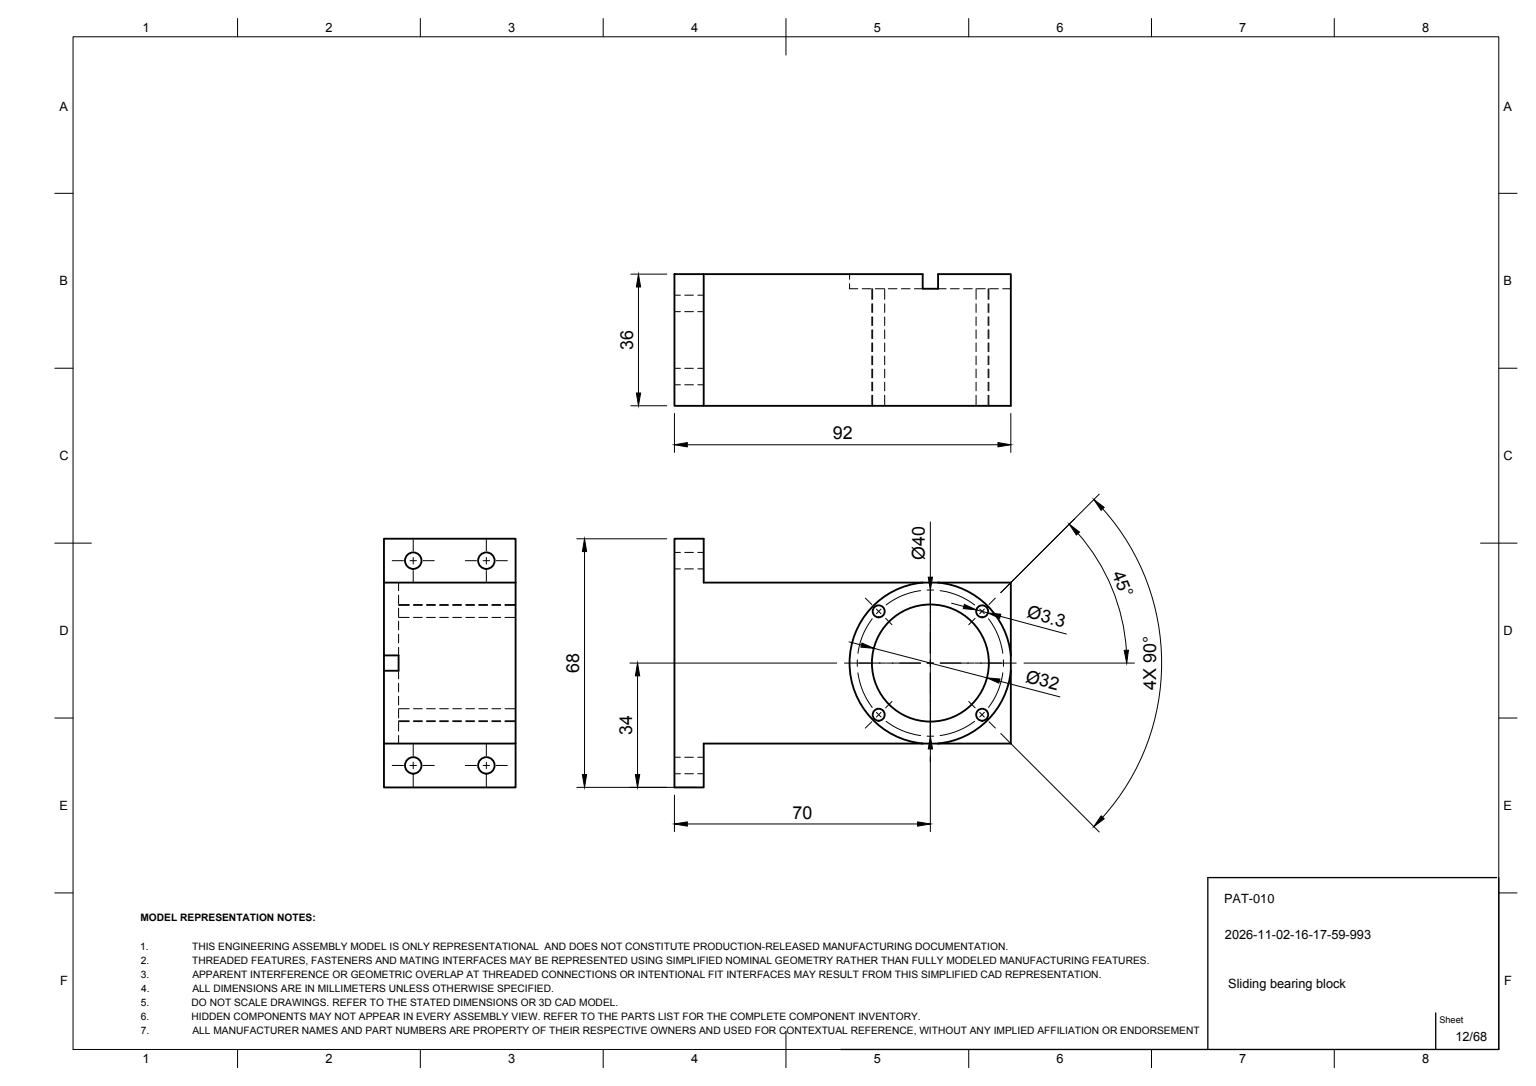
ISO-10303-21;
HEADER;
/* Generated by software containing ST-Developer
 * from STEP Tools, Inc. (www.steptools.com) 
 */

FILE_DESCRIPTION(
/* description */ ('Belt conveyor head drive unit'),
/* implementation_level */ '2;1');

FILE_NAME(
/* name */ 'Sliding bearing block.step',
/* time_stamp */ '2026-10-28T03:26:19-07:00',
/* author */ (''),
/* organization */ (''),
/* preprocessor_version */ 'ST-DEVELOPER v20.2',
/* originating_system */ 'Autodesk Translation Framework v15.17.0.0',
/* authorisation */ '');

FILE_SCHEMA (('AUTOMOTIVE_DESIGN { 1 0 10303 214 3 1 1 }'));
ENDSEC;

DATA;
#10=MECHANICAL_DESIGN_GEOMETRIC_PRESENTATION_REPRESENTATION('',(#854),#27069);
#716=SHAPE_REPRESENTATION_RELATIONSHIP('SRR','None',#27360,#785);
#785=ADVANCED_BREP_SHAPE_REPRESENTATION('',(#939),#27002);
#854=STYLED_ITEM('',(#27797),#939);
#939=MANIFOLD_SOLID_BREP('Body1',#13719);
#1058=FACE_BOUND('',#2593,.T.);
#1059=FACE_BOUND('',#2594,.T.);
#1060=FACE_BOUND('',#2595,.T.);
#1061=FACE_BOUND('',#2596,.T.);
#1062=FACE_BOUND('',#2597,.T.);
#1063=FACE_BOUND('',#2613,.T.);
#1064=FACE_BOUND('',#2614,.T.);
#1065=FACE_BOUND('',#2616,.T.);
#1066=FACE_BOUND('',#2617,.T.);
#1067=FACE_BOUND('',#2621,.T.);
#1068=FACE_BOUND('',#2622,.T.);
#1069=FACE_BOUND('',#2623,.T.);
#1070=FACE_BOUND('',#2624,.T.);
#1071=FACE_BOUND('',#2625,.T.);
#1072=FACE_BOUND('',#2629,.T.);
#1073=FACE_BOUND('',#2630,.T.);
#1074=FACE_BOUND('',#2631,.T.);
#1075=FACE_BOUND('',#2632,.T.);
#1335=PLANE('',#14799);
#1336=PLANE('',#14808);
#1337=PLANE('',#14809);
#1338=PLANE('',#14810);
#1339=PLANE('',#14811);
#1340=PLANE('',#14834);
#1341=PLANE('',#14835);
#1342=PLANE('',#14836);
#1343=PLANE('',#14837);
#1344=PLANE('',#14838);
#1345=PLANE('',#14839);
#1346=PLANE('',#14840);
#1347=PLANE('',#14841);
#1744=FACE_OUTER_BOUND('',#2590,.T.);
#1745=FACE_OUTER_BOUND('',#2591,.T.);
#1746=FACE_OUTER_BOUND('',#2592,.T.);
#1747=FACE_OUTER_BOUND('',#2598,.T.);
#1748=FACE_OUTER_BOUND('',#2599,.T.);
#1749=FACE_OUTER_BOUND('',#2600,.T.);
#1750=FACE_OUTER_BOUND('',#2601,.T.);
#1751=FACE_OUTER_BOUND('',#2602,.T.);
#1752=FACE_OUTER_BOUND('',#2603,.T.);
#1753=FACE_OUTER_BOUND('',#2604,.T.);
#1754=FACE_OUTER_BOUND('',#2605,.T.);
#1755=FACE_OUTER_BOUND('',#2606,.T.);
#1756=FACE_OUTER_BOUND('',#2607,.T.);
#1757=FACE_OUTER_BOUND('',#2608,.T.);
#1758=FACE_OUTER_BOUND('',#2609,.T.);
#1759=FACE_OUTER_BOUND('',#2610,.T.);
#1760=FACE_OUTER_BOUND('',#2611,.T.);
#1761=FACE_OUTER_BOUND('',#2612,.T.);
#1762=FACE_OUTER_BOUND('',#2615,.T.);
#1763=FACE_OUTER_BOUND('',#2618,.T.);
#1764=FACE_OUTER_BOUND('',#2619,.T.);
#1765=FACE_OUTER_BOUND('',#2620,.T.);
#1766=FACE_OUTER_BOUND('',#2626,.T.);
#1767=FACE_OUTER_BOUND('',#2627,.T.);
#1768=FACE_OUTER_BOUND('',#2628,.T.);
#2590=EDGE_LOOP('',(#9456,#9457,#9458,#9459));
#2591=EDGE_LOOP('',(#9460,#9461,#9462,#9463));
#2592=EDGE_LOOP('',(#9464,#9465,#9466,#9467,#9468,#9469));
#2593=EDGE_LOOP('',(#9470));
#2594=EDGE_LOOP('',(#9471));
#2595=EDGE_LOOP('',(#9472));
#2596=EDGE_LOOP('',(#9473));
#2597=EDGE_LOOP('',(#9474));
#2598=EDGE_LOOP('',(#9475,#9476,#9477,#9478));
#2599=EDGE_LOOP('',(#9479,#9480,#9481,#9482,#9483,#9484,#9485,#9486));
#2600=EDGE_LOOP('',(#9487,#9488,#9489,#9490,#9491,#9492,#9493,#9494));
#2601=EDGE_LOOP('',(#9495,#9496,#9497));
#2602=EDGE_LOOP('',(#9498,#9499,#9500));
#2603=EDGE_LOOP('',(#9501,#9502,#9503,#9504));
#2604=EDGE_LOOP('',(#9505,#9506,#9507,#9508));
#2605=EDGE_LOOP('',(#9509,#9510,#9511,#9512));
#2606=EDGE_LOOP('',(#9513,#9514,#9515,#9516));
#2607=EDGE_LOOP('',(#9517,#9518,#9519,#9520));
#2608=EDGE_LOOP('',(#9521,#9522,#9523,#9524));
#2609=EDGE_LOOP('',(#9525,#9526,#9527,#9528));
#2610=EDGE_LOOP('',(#9529,#9530,#9531,#9532));
#2611=EDGE_LOOP('',(#9533,#9534,#9535,#9536));
#2612=EDGE_LOOP('',(#9537,#9538,#9539,#9540));
#2613=EDGE_LOOP('',(#9541));
#2614=EDGE_LOOP('',(#9542));
#2615=EDGE_LOOP('',(#9543,#9544,#9545,#9546));
#2616=EDGE_LOOP('',(#9547));
#2617=EDGE_LOOP('',(#9548));
#2618=EDGE_LOOP('',(#9549,#9550,#9551,#9552));
#2619=EDGE_LOOP('',(#9553,#9554,#9555,#9556));
#2620=EDGE_LOOP('',(#9557,#9558,#9559,#9560,#9561,#9562,#9563,#9564));
#2621=EDGE_LOOP('',(#9565));
#2622=EDGE_LOOP('',(#9566));
#2623=EDGE_LOOP('',(#9567));
#2624=EDGE_LOOP('',(#9568));
#2625=EDGE_LOOP('',(#9569));
#2626=EDGE_LOOP('',(#9570,#9571,#9572,#9573,#9574,#9575,#9576,#9577));
#2627=EDGE_LOOP('',(#9578,#9579,#9580,#9581,#9582,#9583,#9584,#9585));
#2628=EDGE_LOOP('',(#9586,#9587,#9588,#9589));
#2629=EDGE_LOOP('',(#9590));
#2630=EDGE_LOOP('',(#9591));
#2631=EDGE_LOOP('',(#9592));
#2632=EDGE_LOOP('',(#9593));
#3637=LINE('',#21509,#4429);
#3638=LINE('',#21513,#4430);
#3639=LINE('',#21518,#4431);
#3640=LINE('',#21522,#4432);
#3641=LINE('',#21526,#4433);
#3642=LINE('',#21529,#4434);
#3643=LINE('',#21530,#4435);
#3644=LINE('',#21543,#4436);
#3645=LINE('',#21546,#4437);
#3646=LINE('',#21549,#4438);
#3647=LINE('',#21551,#4439);
#3648=LINE('',#21553,#4440);
#3649=LINE('',#21555,#4441);
#3650=LINE('',#21556,#4442);
#3651=LINE('',#21559,#4443);
#3652=LINE('',#21561,#4444);
#3653=LINE('',#21562,#4445);
#3654=LINE('',#21563,#4446);
#3655=LINE('',#21566,#4447);
#3656=LINE('',#21570,#4448);
#3657=LINE('',#21574,#4449);
#3658=LINE('',#21578,#4450);
#3659=LINE('',#21582,#4451);
#3660=LINE('',#21586,#4452);
#3661=LINE('',#21591,#4453);
#3662=LINE('',#21597,#4454);
#3663=LINE('',#21603,#4455);
#3664=LINE('',#21609,#4456);
#3665=LINE('',#21613,#4457);
#3666=LINE('',#21615,#4458);
#3667=LINE('',#21616,#4459);
#3668=LINE('',#21620,#4460);
#3669=LINE('',#21622,#4461);
#3670=LINE('',#21624,#4462);
#3671=LINE('',#21625,#4463);
#3672=LINE('',#21628,#4464);
#3673=LINE('',#21630,#4465);
#3674=LINE('',#21631,#4466);
#3675=LINE('',#21634,#4467);
#3676=LINE('',#21636,#4468);
#3677=LINE('',#21637,#4469);
#3678=LINE('',#21639,#4470);
#3679=LINE('',#21640,#4471);
#3680=LINE('',#21642,#4472);
#3681=LINE('',#21643,#4473);
#4429=VECTOR('',#17037,1.);
#4430=VECTOR('',#17040,1.);
#4431=VECTOR('',#17045,1.);
#4432=VECTOR('',#17048,1.);
#4433=VECTOR('',#17053,1.);
#4434=VECTOR('',#17056,1.);
#4435=VECTOR('',#17057,1.);
#4436=VECTOR('',#17070,1.);
#4437=VECTOR('',#17073,1.);
#4438=VECTOR('',#17076,1.);
#4439=VECTOR('',#17077,1.);
#4440=VECTOR('',#17078,1.);
#4441=VECTOR('',#17079,1.);
#4442=VECTOR('',#17080,1.);
#4443=VECTOR('',#17083,1.);
#4444=VECTOR('',#17084,1.);
#4445=VECTOR('',#17085,1.);
#4446=VECTOR('',#17086,1.);
#4447=VECTOR('',#17091,1.);
#4448=VECTOR('',#17096,0.165);
#4449=VECTOR('',#17101,0.165);
#4450=VECTOR('',#17106,0.164999999999999);
#4451=VECTOR('',#17111,0.164999999999999);
#4452=VECTOR('',#17116,1.6);
#4453=VECTOR('',#17121,0.225);
#4454=VECTOR('',#17128,0.225);
#4455=VECTOR('',#17135,0.225);
#4456=VECTOR('',#17142,0.225);
#4457=VECTOR('',#17147,1.);
#4458=VECTOR('',#17148,1.);
#4459=VECTOR('',#17149,1.);
#4460=VECTOR('',#17152,1.);
#4461=VECTOR('',#17153,1.);
#4462=VECTOR('',#17154,1.);
#4463=VECTOR('',#17155,1.);
#4464=VECTOR('',#17158,1.);
#4465=VECTOR('',#17159,1.);
#4466=VECTOR('',#17160,1.);
#4467=VECTOR('',#17163,1.);
#4468=VECTOR('',#17164,1.);
#4469=VECTOR('',#17165,1.);
#4470=VECTOR('',#17168,1.);
#4471=VECTOR('',#17169,1.);
#4472=VECTOR('',#17172,1.);
#4473=VECTOR('',#17173,1.);
#5192=CIRCLE('',#14794,2.21);
#5193=CIRCLE('',#14795,2.21);
#5194=CIRCLE('',#14797,2.21);
#5195=CIRCLE('',#14798,2.21);
#5196=CIRCLE('',#14800,2.21);
#5197=CIRCLE('',#14801,1.6);
#5198=CIRCLE('',#14802,0.164999999999999);
#5199=CIRCLE('',#14803,0.164999999999999);
#5200=CIRCLE('',#14804,0.165);
#5201=CIRCLE('',#14805,0.165);
#5202=CIRCLE('',#14807,2.21);
#5203=CIRCLE('',#14813,0.165);
#5204=CIRCLE('',#14815,0.165);
#5205=CIRCLE('',#14817,0.164999999999999);
#5206=CIRCLE('',#14819,0.164999999999999);
#5207=CIRCLE('',#14821,1.6);
#5208=CIRCLE('',#14823,0.225);
#5209=CIRCLE('',#14824,0.225);
#5210=CIRCLE('',#14826,0.225);
#5211=CIRCLE('',#14827,0.225);
#5212=CIRCLE('',#14829,0.225);
#5213=CIRCLE('',#14830,0.225);
#5214=CIRCLE('',#14832,0.225);
#5215=CIRCLE('',#14833,0.225);
#6119=VERTEX_POINT('',#21507);
#6120=VERTEX_POINT('',#21508);
#6121=VERTEX_POINT('',#21510);
#6122=VERTEX_POINT('',#21512);
#6123=VERTEX_POINT('',#21516);
#6124=VERTEX_POINT('',#21517);
#6125=VERTEX_POINT('',#21519);
#6126=VERTEX_POINT('',#21521);
#6127=VERTEX_POINT('',#21525);
#6128=VERTEX_POINT('',#21527);
#6129=VERTEX_POINT('',#21531);
#6130=VERTEX_POINT('',#21533);
#6131=VERTEX_POINT('',#21535);
#6132=VERTEX_POINT('',#21537);
#6133=VERTEX_POINT('',#21539);
#6134=VERTEX_POINT('',#21542);
#6135=VERTEX_POINT('',#21544);
#6136=VERTEX_POINT('',#21548);
#6137=VERTEX_POINT('',#21550);
#6138=VERTEX_POINT('',#21552);
#6139=VERTEX_POINT('',#21554);
#6140=VERTEX_POINT('',#21558);
#6141=VERTEX_POINT('',#21560);
#6142=VERTEX_POINT('',#21568);
#6143=VERTEX_POINT('',#21572);
#6144=VERTEX_POINT('',#21576);
#6145=VERTEX_POINT('',#21580);
#6146=VERTEX_POINT('',#21584);
#6147=VERTEX_POINT('',#21588);
#6148=VERTEX_POINT('',#21590);
#6149=VERTEX_POINT('',#21594);
#6150=VERTEX_POINT('',#21596);
#6151=VERTEX_POINT('',#21600);
#6152=VERTEX_POINT('',#21602);
#6153=VERTEX_POINT('',#21606);
#6154=VERTEX_POINT('',#21608);
#6155=VERTEX_POINT('',#21612);
#6156=VERTEX_POINT('',#21614);
#6157=VERTEX_POINT('',#21618);
#6158=VERTEX_POINT('',#21619);
#6159=VERTEX_POINT('',#21621);
#6160=VERTEX_POINT('',#21623);
#6161=VERTEX_POINT('',#21627);
#6162=VERTEX_POINT('',#21629);
#6163=VERTEX_POINT('',#21633);
#6164=VERTEX_POINT('',#21635);
#7420=EDGE_CURVE('',#6119,#6120,#3637,.T.);
#7421=EDGE_CURVE('',#6121,#6119,#5192,.T.);
#7422=EDGE_CURVE('',#6122,#6121,#3638,.T.);
#7423=EDGE_CURVE('',#6120,#6122,#5193,.T.);
#7424=EDGE_CURVE('',#6123,#6124,#3639,.T.);
#7425=EDGE_CURVE('',#6125,#6123,#5194,.T.);
#7426=EDGE_CURVE('',#6126,#6125,#3640,.T.);
#7427=EDGE_CURVE('',#6124,#6126,#5195,.T.);
#7428=EDGE_CURVE('',#6127,#6119,#3641,.T.);
#7429=EDGE_CURVE('',#6127,#6128,#5196,.T.);
#7430=EDGE_CURVE('',#6124,#6128,#3642,.T.);
#7431=EDGE_CURVE('',#6121,#6126,#3643,.T.);
#7432=EDGE_CURVE('',#6129,#6129,#5197,.T.);
#7433=EDGE_CURVE('',#6130,#6130,#5198,.T.);
#7434=EDGE_CURVE('',#6131,#6131,#5199,.T.);
#7435=EDGE_CURVE('',#6132,#6132,#5200,.T.);
#7436=EDGE_CURVE('',#6133,#6133,#5201,.T.);
#7437=EDGE_CURVE('',#6134,#6127,#3644,.T.);
#7438=EDGE_CURVE('',#6135,#6134,#5202,.T.);
#7439=EDGE_CURVE('',#6128,#6135,#3645,.T.);
#7440=EDGE_CURVE('',#6120,#6136,#3646,.T.);
#7441=EDGE_CURVE('',#6137,#6136,#3647,.T.);
#7442=EDGE_CURVE('',#6138,#6137,#3648,.T.);
#7443=EDGE_CURVE('',#6138,#6139,#3649,.T.);
#7444=EDGE_CURVE('',#6139,#6134,#3650,.T.);
#7445=EDGE_CURVE('',#6125,#6140,#3651,.T.);
#7446=EDGE_CURVE('',#6140,#6141,#3652,.T.);
#7447=EDGE_CURVE('',#6141,#6137,#3653,.T.);
#7448=EDGE_CURVE('',#6136,#6122,#3654,.T.);
#7449=EDGE_CURVE('',#6123,#6140,#3655,.T.);
#7450=EDGE_CURVE('',#6142,#6142,#5203,.T.);
#7451=EDGE_CURVE('',#6142,#6133,#3656,.T.);
#7452=EDGE_CURVE('',#6143,#6143,#5204,.T.);
#7453=EDGE_CURVE('',#6143,#6132,#3657,.T.);
#7454=EDGE_CURVE('',#6144,#6144,#5205,.T.);
#7455=EDGE_CURVE('',#6144,#6131,#3658,.T.);
#7456=EDGE_CURVE('',#6145,#6145,#5206,.T.);
#7457=EDGE_CURVE('',#6145,#6130,#3659,.T.);
#7458=EDGE_CURVE('',#6146,#6146,#5207,.T.);
#7459=EDGE_CURVE('',#6146,#6129,#3660,.T.);
#7460=EDGE_CURVE('',#6147,#6147,#5208,.T.);
#7461=EDGE_CURVE('',#6147,#6148,#3661,.T.);
#7462=EDGE_CURVE('',#6148,#6148,#5209,.T.);
#7463=EDGE_CURVE('',#6149,#6149,#5210,.T.);
#7464=EDGE_CURVE('',#6149,#6150,#3662,.T.);
#7465=EDGE_CURVE('',#6150,#6150,#5211,.T.);
#7466=EDGE_CURVE('',#6151,#6151,#5212,.T.);
#7467=EDGE_CURVE('',#6151,#6152,#3663,.T.);
#7468=EDGE_CURVE('',#6152,#6152,#5213,.T.);
#7469=EDGE_CURVE('',#6153,#6153,#5214,.T.);
#7470=EDGE_CURVE('',#6153,#6154,#3664,.T.);
#7471=EDGE_CURVE('',#6154,#6154,#5215,.T.);
#7472=EDGE_CURVE('',#6155,#6138,#3665,.T.);
#7473=EDGE_CURVE('',#6155,#6156,#3666,.T.);
#7474=EDGE_CURVE('',#6139,#6156,#3667,.T.);
#7475=EDGE_CURVE('',#6157,#6158,#3668,.T.);
#7476=EDGE_CURVE('',#6159,#6157,#3669,.T.);
#7477=EDGE_CURVE('',#6160,#6159,#3670,.T.);
#7478=EDGE_CURVE('',#6158,#6160,#3671,.T.);
#7479=EDGE_CURVE('',#6160,#6161,#3672,.T.);
#7480=EDGE_CURVE('',#6162,#6159,#3673,.T.);
#7481=EDGE_CURVE('',#6161,#6162,#3674,.T.);
#7482=EDGE_CURVE('',#6163,#6155,#3675,.T.);
#7483=EDGE_CURVE('',#6163,#6164,#3676,.T.);
#7484=EDGE_CURVE('',#6156,#6164,#3677,.T.);
#7485=EDGE_CURVE('',#6158,#6141,#3678,.T.);
#7486=EDGE_CURVE('',#6161,#6163,#3679,.T.);
#7487=EDGE_CURVE('',#6164,#6162,#3680,.T.);
#7488=EDGE_CURVE('',#6157,#6135,#3681,.T.);
#9456=ORIENTED_EDGE('',*,*,#7420,.F.);
#9457=ORIENTED_EDGE('',*,*,#7421,.F.);
#9458=ORIENTED_EDGE('',*,*,#7422,.F.);
#9459=ORIENTED_EDGE('',*,*,#7423,.F.);
#9460=ORIENTED_EDGE('',*,*,#7424,.F.);
#9461=ORIENTED_EDGE('',*,*,#7425,.F.);
#9462=ORIENTED_EDGE('',*,*,#7426,.F.);
#9463=ORIENTED_EDGE('',*,*,#7427,.F.);
#9464=ORIENTED_EDGE('',*,*,#7428,.F.);
#9465=ORIENTED_EDGE('',*,*,#7429,.T.);
#9466=ORIENTED_EDGE('',*,*,#7430,.F.);
#9467=ORIENTED_EDGE('',*,*,#7427,.T.);
#9468=ORIENTED_EDGE('',*,*,#7431,.F.);
#9469=ORIENTED_EDGE('',*,*,#7421,.T.);
#9470=ORIENTED_EDGE('',*,*,#7432,.F.);
#9471=ORIENTED_EDGE('',*,*,#7433,.F.);
#9472=ORIENTED_EDGE('',*,*,#7434,.F.);
#9473=ORIENTED_EDGE('',*,*,#7435,.F.);
#9474=ORIENTED_EDGE('',*,*,#7436,.F.);
#9475=ORIENTED_EDGE('',*,*,#7437,.F.);
#9476=ORIENTED_EDGE('',*,*,#7438,.F.);
#9477=ORIENTED_EDGE('',*,*,#7439,.F.);
#9478=ORIENTED_EDGE('',*,*,#7429,.F.);
#9479=ORIENTED_EDGE('',*,*,#7437,.T.);
#9480=ORIENTED_EDGE('',*,*,#7428,.T.);
#9481=ORIENTED_EDGE('',*,*,#7420,.T.);
#9482=ORIENTED_EDGE('',*,*,#7440,.T.);
#9483=ORIENTED_EDGE('',*,*,#7441,.F.);
#9484=ORIENTED_EDGE('',*,*,#7442,.F.);
#9485=ORIENTED_EDGE('',*,*,#7443,.T.);
#9486=ORIENTED_EDGE('',*,*,#7444,.T.);
#9487=ORIENTED_EDGE('',*,*,#7422,.T.);
#9488=ORIENTED_EDGE('',*,*,#7431,.T.);
#9489=ORIENTED_EDGE('',*,*,#7426,.T.);
#9490=ORIENTED_EDGE('',*,*,#7445,.T.);
#9491=ORIENTED_EDGE('',*,*,#7446,.T.);
#9492=ORIENTED_EDGE('',*,*,#7447,.T.);
#9493=ORIENTED_EDGE('',*,*,#7441,.T.);
#9494=ORIENTED_EDGE('',*,*,#7448,.T.);
#9495=ORIENTED_EDGE('',*,*,#7423,.T.);
#9496=ORIENTED_EDGE('',*,*,#7448,.F.);
#9497=ORIENTED_EDGE('',*,*,#7440,.F.);
#9498=ORIENTED_EDGE('',*,*,#7425,.T.);
#9499=ORIENTED_EDGE('',*,*,#7449,.T.);
#9500=ORIENTED_EDGE('',*,*,#7445,.F.);
#9501=ORIENTED_EDGE('',*,*,#7450,.F.);
#9502=ORIENTED_EDGE('',*,*,#7451,.T.);
#9503=ORIENTED_EDGE('',*,*,#7436,.T.);
#9504=ORIENTED_EDGE('',*,*,#7451,.F.);
#9505=ORIENTED_EDGE('',*,*,#7452,.F.);
#9506=ORIENTED_EDGE('',*,*,#7453,.T.);
#9507=ORIENTED_EDGE('',*,*,#7435,.T.);
#9508=ORIENTED_EDGE('',*,*,#7453,.F.);
#9509=ORIENTED_EDGE('',*,*,#7454,.F.);
#9510=ORIENTED_EDGE('',*,*,#7455,.T.);
#9511=ORIENTED_EDGE('',*,*,#7434,.T.);
#9512=ORIENTED_EDGE('',*,*,#7455,.F.);
#9513=ORIENTED_EDGE('',*,*,#7456,.F.);
#9514=ORIENTED_EDGE('',*,*,#7457,.T.);
#9515=ORIENTED_EDGE('',*,*,#7433,.T.);
#9516=ORIENTED_EDGE('',*,*,#7457,.F.);
#9517=ORIENTED_EDGE('',*,*,#7458,.F.);
#9518=ORIENTED_EDGE('',*,*,#7459,.T.);
#9519=ORIENTED_EDGE('',*,*,#7432,.T.);
#9520=ORIENTED_EDGE('',*,*,#7459,.F.);
#9521=ORIENTED_EDGE('',*,*,#7460,.F.);
#9522=ORIENTED_EDGE('',*,*,#7461,.T.);
#9523=ORIENTED_EDGE('',*,*,#7462,.F.);
#9524=ORIENTED_EDGE('',*,*,#7461,.F.);
#9525=ORIENTED_EDGE('',*,*,#7463,.F.);
#9526=ORIENTED_EDGE('',*,*,#7464,.T.);
#9527=ORIENTED_EDGE('',*,*,#7465,.F.);
#9528=ORIENTED_EDGE('',*,*,#7464,.F.);
#9529=ORIENTED_EDGE('',*,*,#7466,.F.);
#9530=ORIENTED_EDGE('',*,*,#7467,.T.);
#9531=ORIENTED_EDGE('',*,*,#7468,.F.);
#9532=ORIENTED_EDGE('',*,*,#7467,.F.);
#9533=ORIENTED_EDGE('',*,*,#7469,.F.);
#9534=ORIENTED_EDGE('',*,*,#7470,.T.);
#9535=ORIENTED_EDGE('',*,*,#7471,.F.);
#9536=ORIENTED_EDGE('',*,*,#7470,.F.);
#9537=ORIENTED_EDGE('',*,*,#7443,.F.);
#9538=ORIENTED_EDGE('',*,*,#7472,.F.);
#9539=ORIENTED_EDGE('',*,*,#7473,.T.);
#9540=ORIENTED_EDGE('',*,*,#7474,.F.);
#9541=ORIENTED_EDGE('',*,*,#7462,.T.);
#9542=ORIENTED_EDGE('',*,*,#7471,.T.);
#9543=ORIENTED_EDGE('',*,*,#7475,.F.);
#9544=ORIENTED_EDGE('',*,*,#7476,.F.);
#9545=ORIENTED_EDGE('',*,*,#7477,.F.);
#9546=ORIENTED_EDGE('',*,*,#7478,.F.);
#9547=ORIENTED_EDGE('',*,*,#7465,.T.);
#9548=ORIENTED_EDGE('',*,*,#7468,.T.);
#9549=ORIENTED_EDGE('',*,*,#7479,.F.);
#9550=ORIENTED_EDGE('',*,*,#7477,.T.);
#9551=ORIENTED_EDGE('',*,*,#7480,.F.);
#9552=ORIENTED_EDGE('',*,*,#7481,.F.);
#9553=ORIENTED_EDGE('',*,*,#7482,.F.);
#9554=ORIENTED_EDGE('',*,*,#7483,.T.);
#9555=ORIENTED_EDGE('',*,*,#7484,.F.);
#9556=ORIENTED_EDGE('',*,*,#7473,.F.);
#9557=ORIENTED_EDGE('',*,*,#7442,.T.);
#9558=ORIENTED_EDGE('',*,*,#7447,.F.);
#9559=ORIENTED_EDGE('',*,*,#7485,.F.);
#9560=ORIENTED_EDGE('',*,*,#7478,.T.);
#9561=ORIENTED_EDGE('',*,*,#7479,.T.);
#9562=ORIENTED_EDGE('',*,*,#7486,.T.);
#9563=ORIENTED_EDGE('',*,*,#7482,.T.);
#9564=ORIENTED_EDGE('',*,*,#7472,.T.);
#9565=ORIENTED_EDGE('',*,*,#7458,.T.);
#9566=ORIENTED_EDGE('',*,*,#7456,.T.);
#9567=ORIENTED_EDGE('',*,*,#7454,.T.);
#9568=ORIENTED_EDGE('',*,*,#7452,.T.);
#9569=ORIENTED_EDGE('',*,*,#7450,.T.);
#9570=ORIENTED_EDGE('',*,*,#7438,.T.);
#9571=ORIENTED_EDGE('',*,*,#7444,.F.);
#9572=ORIENTED_EDGE('',*,*,#7474,.T.);
#9573=ORIENTED_EDGE('',*,*,#7484,.T.);
#9574=ORIENTED_EDGE('',*,*,#7487,.T.);
#9575=ORIENTED_EDGE('',*,*,#7480,.T.);
#9576=ORIENTED_EDGE('',*,*,#7476,.T.);
#9577=ORIENTED_EDGE('',*,*,#7488,.T.);
#9578=ORIENTED_EDGE('',*,*,#7439,.T.);
#9579=ORIENTED_EDGE('',*,*,#7488,.F.);
#9580=ORIENTED_EDGE('',*,*,#7475,.T.);
#9581=ORIENTED_EDGE('',*,*,#7485,.T.);
#9582=ORIENTED_EDGE('',*,*,#7446,.F.);
#9583=ORIENTED_EDGE('',*,*,#7449,.F.);
#9584=ORIENTED_EDGE('',*,*,#7424,.T.);
#9585=ORIENTED_EDGE('',*,*,#7430,.T.);
#9586=ORIENTED_EDGE('',*,*,#7487,.F.);
#9587=ORIENTED_EDGE('',*,*,#7483,.F.);
#9588=ORIENTED_EDGE('',*,*,#7486,.F.);
#9589=ORIENTED_EDGE('',*,*,#7481,.T.);
#9590=ORIENTED_EDGE('',*,*,#7460,.T.);
#9591=ORIENTED_EDGE('',*,*,#7463,.T.);
#9592=ORIENTED_EDGE('',*,*,#7466,.T.);
#9593=ORIENTED_EDGE('',*,*,#7469,.T.);
#12585=CYLINDRICAL_SURFACE('',#14793,2.21);
#12586=CYLINDRICAL_SURFACE('',#14796,2.21);
#12587=CYLINDRICAL_SURFACE('',#14806,2.21);
#12588=CYLINDRICAL_SURFACE('',#14812,0.165);
#12589=CYLINDRICAL_SURFACE('',#14814,0.165);
#12590=CYLINDRICAL_SURFACE('',#14816,0.164999999999999);
#12591=CYLINDRICAL_SURFACE('',#14818,0.164999999999999);
#12592=CYLINDRICAL_SURFACE('',#14820,1.6);
#12593=CYLINDRICAL_SURFACE('',#14822,0.225);
#12594=CYLINDRICAL_SURFACE('',#14825,0.225);
#12595=CYLINDRICAL_SURFACE('',#14828,0.225);
#12596=CYLINDRICAL_SURFACE('',#14831,0.225);
#13023=ADVANCED_FACE('',(#1744),#12585,.F.);
#13024=ADVANCED_FACE('',(#1745),#12586,.F.);
#13025=ADVANCED_FACE('',(#1746,#1058,#1059,#1060,#1061,#1062),#1335,.T.);
#13026=ADVANCED_FACE('',(#1747),#12587,.F.);
#13027=ADVANCED_FACE('',(#1748),#1336,.T.);
#13028=ADVANCED_FACE('',(#1749),#1337,.T.);
#13029=ADVANCED_FACE('',(#1750),#1338,.T.);
#13030=ADVANCED_FACE('',(#1751),#1339,.T.);
#13031=ADVANCED_FACE('',(#1752),#12588,.F.);
#13032=ADVANCED_FACE('',(#1753),#12589,.F.);
#13033=ADVANCED_FACE('',(#1754),#12590,.F.);
#13034=ADVANCED_FACE('',(#1755),#12591,.F.);
#13035=ADVANCED_FACE('',(#1756),#12592,.F.);
#13036=ADVANCED_FACE('',(#1757),#12593,.F.);
#13037=ADVANCED_FACE('',(#1758),#12594,.F.);
#13038=ADVANCED_FACE('',(#1759),#12595,.F.);
#13039=ADVANCED_FACE('',(#1760),#12596,.F.);
#13040=ADVANCED_FACE('',(#1761,#1063,#1064),#1340,.T.);
#13041=ADVANCED_FACE('',(#1762,#1065,#1066),#1341,.T.);
#13042=ADVANCED_FACE('',(#1763),#1342,.T.);
#13043=ADVANCED_FACE('',(#1764),#1343,.T.);
#13044=ADVANCED_FACE('',(#1765,#1067,#1068,#1069,#1070,#1071),#1344,.T.);
#13045=ADVANCED_FACE('',(#1766),#1345,.T.);
#13046=ADVANCED_FACE('',(#1767),#1346,.T.);
#13047=ADVANCED_FACE('',(#1768,#1072,#1073,#1074,#1075),#1347,.F.);
#13719=CLOSED_SHELL('',(#13023,#13024,#13025,#13026,#13027,#13028,#13029,
#13030,#13031,#13032,#13033,#13034,#13035,#13036,#13037,#13038,#13039,#13040,
#13041,#13042,#13043,#13044,#13045,#13046,#13047));
#14792=AXIS2_PLACEMENT_3D('',#21505,#17033,#17034);
#14793=AXIS2_PLACEMENT_3D('',#21506,#17035,#17036);
#14794=AXIS2_PLACEMENT_3D('',#21511,#17038,#17039);
#14795=AXIS2_PLACEMENT_3D('',#21514,#17041,#17042);
#14796=AXIS2_PLACEMENT_3D('',#21515,#17043,#17044);
#14797=AXIS2_PLACEMENT_3D('',#21520,#17046,#17047);
#14798=AXIS2_PLACEMENT_3D('',#21523,#17049,#17050);
#14799=AXIS2_PLACEMENT_3D('',#21524,#17051,#17052);
#14800=AXIS2_PLACEMENT_3D('',#21528,#17054,#17055);
#14801=AXIS2_PLACEMENT_3D('',#21532,#17058,#17059);
#14802=AXIS2_PLACEMENT_3D('',#21534,#17060,#17061);
#14803=AXIS2_PLACEMENT_3D('',#21536,#17062,#17063);
#14804=AXIS2_PLACEMENT_3D('',#21538,#17064,#17065);
#14805=AXIS2_PLACEMENT_3D('',#21540,#17066,#17067);
#14806=AXIS2_PLACEMENT_3D('',#21541,#17068,#17069);
#14807=AXIS2_PLACEMENT_3D('',#21545,#17071,#17072);
#14808=AXIS2_PLACEMENT_3D('',#21547,#17074,#17075);
#14809=AXIS2_PLACEMENT_3D('',#21557,#17081,#17082);
#14810=AXIS2_PLACEMENT_3D('',#21564,#17087,#17088);
#14811=AXIS2_PLACEMENT_3D('',#21565,#17089,#17090);
#14812=AXIS2_PLACEMENT_3D('',#21567,#17092,#17093);
#14813=AXIS2_PLACEMENT_3D('',#21569,#17094,#17095);
#14814=AXIS2_PLACEMENT_3D('',#21571,#17097,#17098);
#14815=AXIS2_PLACEMENT_3D('',#21573,#17099,#17100);
#14816=AXIS2_PLACEMENT_3D('',#21575,#17102,#17103);
#14817=AXIS2_PLACEMENT_3D('',#21577,#17104,#17105);
#14818=AXIS2_PLACEMENT_3D('',#21579,#17107,#17108);
#14819=AXIS2_PLACEMENT_3D('',#21581,#17109,#17110);
#14820=AXIS2_PLACEMENT_3D('',#21583,#17112,#17113);
#14821=AXIS2_PLACEMENT_3D('',#21585,#17114,#17115);
#14822=AXIS2_PLACEMENT_3D('',#21587,#17117,#17118);
#14823=AXIS2_PLACEMENT_3D('',#21589,#17119,#17120);
#14824=AXIS2_PLACEMENT_3D('',#21592,#17122,#17123);
#14825=AXIS2_PLACEMENT_3D('',#21593,#17124,#17125);
#14826=AXIS2_PLACEMENT_3D('',#21595,#17126,#17127);
#14827=AXIS2_PLACEMENT_3D('',#21598,#17129,#17130);
#14828=AXIS2_PLACEMENT_3D('',#21599,#17131,#17132);
#14829=AXIS2_PLACEMENT_3D('',#21601,#17133,#17134);
#14830=AXIS2_PLACEMENT_3D('',#21604,#17136,#17137);
#14831=AXIS2_PLACEMENT_3D('',#21605,#17138,#17139);
#14832=AXIS2_PLACEMENT_3D('',#21607,#17140,#17141);
#14833=AXIS2_PLACEMENT_3D('',#21610,#17143,#17144);
#14834=AXIS2_PLACEMENT_3D('',#21611,#17145,#17146);
#14835=AXIS2_PLACEMENT_3D('',#21617,#17150,#17151);
#14836=AXIS2_PLACEMENT_3D('',#21626,#17156,#17157);
#14837=AXIS2_PLACEMENT_3D('',#21632,#17161,#17162);
#14838=AXIS2_PLACEMENT_3D('',#21638,#17166,#17167);
#14839=AXIS2_PLACEMENT_3D('',#21641,#17170,#17171);
#14840=AXIS2_PLACEMENT_3D('',#21644,#17174,#17175);
#14841=AXIS2_PLACEMENT_3D('',#21645,#17176,#17177);
#17033=DIRECTION('axis',(0.,0.,1.));
#17034=DIRECTION('refdir',(1.,0.,0.));
#17035=DIRECTION('center_axis',(0.,1.,0.));
#17036=DIRECTION('ref_axis',(1.,0.,0.));
#17037=DIRECTION('',(0.,1.,0.));
#17038=DIRECTION('center_axis',(0.,1.,0.));
#17039=DIRECTION('ref_axis',(1.,0.,0.));
#17040=DIRECTION('',(0.,-1.,0.));
#17041=DIRECTION('center_axis',(0.,-1.,0.));
#17042=DIRECTION('ref_axis',(1.,0.,0.));
#17043=DIRECTION('center_axis',(0.,1.,0.));
#17044=DIRECTION('ref_axis',(1.,0.,0.));
#17045=DIRECTION('',(0.,-1.,0.));
#17046=DIRECTION('center_axis',(0.,-1.,0.));
#17047=DIRECTION('ref_axis',(1.,0.,0.));
#17048=DIRECTION('',(0.,1.,0.));
#17049=DIRECTION('center_axis',(0.,1.,0.));
#17050=DIRECTION('ref_axis',(1.,0.,0.));
#17051=DIRECTION('center_axis',(0.,1.,0.));
#17052=DIRECTION('ref_axis',(1.,0.,0.));
#17053=DIRECTION('',(0.,0.,1.));
#17054=DIRECTION('center_axis',(0.,1.,0.));
#17055=DIRECTION('ref_axis',(1.,0.,0.));
#17056=DIRECTION('',(0.,0.,-1.));
#17057=DIRECTION('',(-1.,0.,0.));
#17058=DIRECTION('center_axis',(0.,1.,0.));
#17059=DIRECTION('ref_axis',(1.,0.,0.));
#17060=DIRECTION('center_axis',(0.,1.,0.));
#17061=DIRECTION('ref_axis',(1.,0.,0.));
#17062=DIRECTION('center_axis',(0.,1.,0.));
#17063=DIRECTION('ref_axis',(1.,0.,0.));
#17064=DIRECTION('center_axis',(0.,1.,0.));
#17065=DIRECTION('ref_axis',(1.,0.,0.));
#17066=DIRECTION('center_axis',(0.,1.,0.));
#17067=DIRECTION('ref_axis',(1.,0.,0.));
#17068=DIRECTION('center_axis',(0.,1.,0.));
#17069=DIRECTION('ref_axis',(1.,0.,0.));
#17070=DIRECTION('',(0.,-1.,0.));
#17071=DIRECTION('center_axis',(0.,-1.,0.));
#17072=DIRECTION('ref_axis',(1.,0.,0.));
#17073=DIRECTION('',(0.,1.,0.));
#17074=DIRECTION('center_axis',(1.,0.,0.));
#17075=DIRECTION('ref_axis',(0.,1.,0.));
#17076=DIRECTION('',(0.,0.,1.));
#17077=DIRECTION('',(0.,1.,0.));
#17078=DIRECTION('',(0.,0.,1.));
#17079=DIRECTION('',(0.,1.,0.));
#17080=DIRECTION('',(0.,0.,1.));
#17081=DIRECTION('center_axis',(0.,0.,1.));
#17082=DIRECTION('ref_axis',(1.,0.,0.));
#17083=DIRECTION('',(-1.,0.,0.));
#17084=DIRECTION('',(0.,-1.,0.));
#17085=DIRECTION('',(1.,0.,0.));
#17086=DIRECTION('',(-1.,0.,0.));
#17087=DIRECTION('center_axis',(0.,1.,0.));
#17088=DIRECTION('ref_axis',(-1.,0.,0.));
#17089=DIRECTION('center_axis',(0.,1.,0.));
#17090=DIRECTION('ref_axis',(-1.,0.,0.));
#17091=DIRECTION('',(0.,0.,1.));
#17092=DIRECTION('center_axis',(0.,1.,0.));
#17093=DIRECTION('ref_axis',(1.,0.,0.));
#17094=DIRECTION('center_axis',(0.,1.,0.));
#17095=DIRECTION('ref_axis',(1.,0.,0.));
#17096=DIRECTION('',(0.,1.,0.));
#17097=DIRECTION('center_axis',(0.,1.,0.));
#17098=DIRECTION('ref_axis',(1.,0.,0.));
#17099=DIRECTION('center_axis',(0.,1.,0.));
#17100=DIRECTION('ref_axis',(1.,0.,0.));
#17101=DIRECTION('',(0.,1.,0.));
#17102=DIRECTION('center_axis',(0.,1.,0.));
#17103=DIRECTION('ref_axis',(1.,0.,0.));
#17104=DIRECTION('center_axis',(0.,1.,0.));
#17105=DIRECTION('ref_axis',(1.,0.,0.));
#17106=DIRECTION('',(0.,1.,0.));
#17107=DIRECTION('center_axis',(0.,1.,0.));
#17108=DIRECTION('ref_axis',(1.,0.,0.));
#17109=DIRECTION('center_axis',(0.,1.,0.));
#17110=DIRECTION('ref_axis',(1.,0.,0.));
#17111=DIRECTION('',(0.,1.,0.));
#17112=DIRECTION('center_axis',(0.,1.,0.));
#17113=DIRECTION('ref_axis',(1.,0.,0.));
#17114=DIRECTION('center_axis',(0.,1.,0.));
#17115=DIRECTION('ref_axis',(1.,0.,0.));
#17116=DIRECTION('',(0.,1.,0.));
#17117=DIRECTION('center_axis',(0.,0.,1.));
#17118=DIRECTION('ref_axis',(1.,0.,0.));
#17119=DIRECTION('center_axis',(0.,0.,1.));
#17120=DIRECTION('ref_axis',(1.,0.,0.));
#17121=DIRECTION('',(0.,0.,1.));
#17122=DIRECTION('center_axis',(0.,0.,-1.));
#17123=DIRECTION('ref_axis',(1.,0.,0.));
#17124=DIRECTION('center_axis',(0.,0.,1.));
#17125=DIRECTION('ref_axis',(1.,0.,0.));
#17126=DIRECTION('center_axis',(0.,0.,1.));
#17127=DIRECTION('ref_axis',(1.,0.,0.));
#17128=DIRECTION('',(0.,0.,1.));
#17129=DIRECTION('center_axis',(0.,0.,-1.));
#17130=DIRECTION('ref_axis',(1.,0.,0.));
#17131=DIRECTION('center_axis',(0.,0.,1.));
#17132=DIRECTION('ref_axis',(1.,0.,0.));
#17133=DIRECTION('center_axis',(0.,0.,1.));
#17134=DIRECTION('ref_axis',(1.,0.,0.));
#17135=DIRECTION('',(0.,0.,1.));
#17136=DIRECTION('center_axis',(0.,0.,-1.));
#17137=DIRECTION('ref_axis',(1.,0.,0.));
#17138=DIRECTION('center_axis',(0.,0.,1.));
#17139=DIRECTION('ref_axis',(1.,0.,0.));
#17140=DIRECTION('center_axis',(0.,0.,1.));
#17141=DIRECTION('ref_axis',(1.,0.,0.));
#17142=DIRECTION('',(0.,0.,1.));
#17143=DIRECTION('center_axis',(0.,0.,-1.));
#17144=DIRECTION('ref_axis',(1.,0.,0.));
#17145=DIRECTION('center_axis',(0.,0.,1.));
#17146=DIRECTION('ref_axis',(1.,0.,0.));
#17147=DIRECTION('',(-1.,0.,0.));
#17148=DIRECTION('',(0.,1.,0.));
#17149=DIRECTION('',(1.,0.,0.));
#17150=DIRECTION('center_axis',(0.,0.,1.));
#17151=DIRECTION('ref_axis',(1.,0.,0.));
#17152=DIRECTION('',(0.,-1.,0.));
#17153=DIRECTION('',(1.,0.,0.));
#17154=DIRECTION('',(0.,1.,0.));
#17155=DIRECTION('',(-1.,0.,0.));
#17156=DIRECTION('center_axis',(-1.,0.,0.));
#17157=DIRECTION('ref_axis',(0.,0.,1.));
#17158=DIRECTION('',(0.,0.,-1.));
#17159=DIRECTION('',(0.,0.,1.));
#17160=DIRECTION('',(0.,1.,0.));
#17161=DIRECTION('center_axis',(1.,0.,0.));
#17162=DIRECTION('ref_axis',(0.,0.,-1.));
#17163=DIRECTION('',(0.,0.,1.));
#17164=DIRECTION('',(0.,1.,0.));
#17165=DIRECTION('',(0.,0.,-1.));
#17166=DIRECTION('center_axis',(0.,-1.,0.));
#17167=DIRECTION('ref_axis',(1.,0.,0.));
#17168=DIRECTION('',(0.,0.,1.));
#17169=DIRECTION('',(1.,0.,0.));
#17170=DIRECTION('center_axis',(0.,1.,0.));
#17171=DIRECTION('ref_axis',(-1.,0.,0.));
#17172=DIRECTION('',(-1.,0.,0.));
#17173=DIRECTION('',(0.,0.,1.));
#17174=DIRECTION('center_axis',(-1.,0.,0.));
#17175=DIRECTION('ref_axis',(0.,-1.,0.));
#17176=DIRECTION('center_axis',(0.,0.,1.));
#17177=DIRECTION('ref_axis',(1.,0.,0.));
#21505=CARTESIAN_POINT('',(0.,0.,0.));
#21506=CARTESIAN_POINT('Origin',(6.97091003018116,1.4,7.));
#21507=CARTESIAN_POINT('',(9.17091003018116,1.4,7.21));
#21508=CARTESIAN_POINT('',(9.17091003018116,1.8,7.21));
#21509=CARTESIAN_POINT('',(9.17091003018116,1.4,7.21));
#21510=CARTESIAN_POINT('',(7.18091003018115,1.4,9.2));
#21511=CARTESIAN_POINT('Origin',(6.97091003018116,1.4,7.));
#21512=CARTESIAN_POINT('',(7.18091003018115,1.8,9.2));
#21513=CARTESIAN_POINT('',(7.18091003018115,1.4,9.2));
#21514=CARTESIAN_POINT('Origin',(6.97091003018116,1.8,7.));
#21515=CARTESIAN_POINT('Origin',(6.97091003018116,1.4,7.));
#21516=CARTESIAN_POINT('',(4.77091003018116,1.8,7.21));
#21517=CARTESIAN_POINT('',(4.77091003018116,1.4,7.21));
#21518=CARTESIAN_POINT('',(4.77091003018116,1.4,7.21));
#21519=CARTESIAN_POINT('',(6.76091003018117,1.8,9.2));
#21520=CARTESIAN_POINT('Origin',(6.97091003018116,1.8,7.));
#21521=CARTESIAN_POINT('',(6.76091003018117,1.4,9.2));
#21522=CARTESIAN_POINT('',(6.76091003018117,1.4,9.2));
#21523=CARTESIAN_POINT('Origin',(6.97091003018116,1.4,7.));
#21524=CARTESIAN_POINT('Origin',(6.97091003018116,1.4,7.));
#21525=CARTESIAN_POINT('',(9.17091003018116,1.4,6.79));
#21526=CARTESIAN_POINT('',(9.17091003018116,1.4,3.5));
#21527=CARTESIAN_POINT('',(4.77091003018116,1.4,6.79));
#21528=CARTESIAN_POINT('Origin',(6.97091003018116,1.4,7.));
#21529=CARTESIAN_POINT('',(4.77091003018116,1.4,3.5));
#21530=CARTESIAN_POINT('',(6.97091003018116,1.4,9.2));
#21531=CARTESIAN_POINT('',(5.37091003018116,1.4,7.));
#21532=CARTESIAN_POINT('Origin',(6.97091003018116,1.4,7.));
#21533=CARTESIAN_POINT('',(8.22012359255425,1.4,5.58578643762691));
#21534=CARTESIAN_POINT('Origin',(8.38512359255425,1.4,5.58578643762691));
#21535=CARTESIAN_POINT('',(8.22012359255425,1.4,8.4142135623731));
#21536=CARTESIAN_POINT('Origin',(8.38512359255425,1.4,8.4142135623731));
#21537=CARTESIAN_POINT('',(5.39169646780806,1.4,8.4142135623731));
#21538=CARTESIAN_POINT('Origin',(5.55669646780806,1.4,8.4142135623731));
#21539=CARTESIAN_POINT('',(5.39169646780806,1.4,5.58578643762691));
#21540=CARTESIAN_POINT('Origin',(5.55669646780806,1.4,5.58578643762691));
#21541=CARTESIAN_POINT('Origin',(6.97091003018116,1.4,7.));
#21542=CARTESIAN_POINT('',(9.17091003018116,1.8,6.79));
#21543=CARTESIAN_POINT('',(9.17091003018116,1.4,6.79));
#21544=CARTESIAN_POINT('',(4.77091003018116,1.8,6.79));
#21545=CARTESIAN_POINT('Origin',(6.97091003018116,1.8,7.));
#21546=CARTESIAN_POINT('',(4.77091003018116,1.4,6.79));
#21547=CARTESIAN_POINT('Origin',(9.17091003018116,-1.8,0.));
#21548=CARTESIAN_POINT('',(9.17091003018116,1.8,9.2));
#21549=CARTESIAN_POINT('',(9.17091003018116,1.8,0.));
#21550=CARTESIAN_POINT('',(9.17091003018116,-1.8,9.2));
#21551=CARTESIAN_POINT('',(9.17091003018116,-1.8,9.2));
#21552=CARTESIAN_POINT('',(9.17091003018116,-1.8,0.8));
#21553=CARTESIAN_POINT('',(9.17091003018116,-1.8,0.));
#21554=CARTESIAN_POINT('',(9.17091003018116,1.8,0.8));
#21555=CARTESIAN_POINT('',(9.17091003018116,-1.8,0.8));
#21556=CARTESIAN_POINT('',(9.17091003018116,1.8,0.));
#21557=CARTESIAN_POINT('Origin',(6.97091003018116,0.,9.2));
#21558=CARTESIAN_POINT('',(4.77091003018116,1.8,9.2));
#21559=CARTESIAN_POINT('',(9.17091003018116,1.8,9.2));
#21560=CARTESIAN_POINT('',(4.77091003018116,-1.8,9.2));
#21561=CARTESIAN_POINT('',(4.77091003018116,1.8,9.2));
#21562=CARTESIAN_POINT('',(4.77091003018116,-1.8,9.2));
#21563=CARTESIAN_POINT('',(9.17091003018116,1.8,9.2));
#21564=CARTESIAN_POINT('Origin',(9.17091003018116,1.8,0.));
#21565=CARTESIAN_POINT('Origin',(9.17091003018116,1.8,0.));
#21566=CARTESIAN_POINT('',(4.77091003018116,1.8,0.));
#21567=CARTESIAN_POINT('Origin',(5.55669646780806,-1.9,5.58578643762691));
#21568=CARTESIAN_POINT('',(5.39169646780806,-1.8,5.58578643762691));
#21569=CARTESIAN_POINT('Origin',(5.55669646780806,-1.8,5.58578643762691));
#21570=CARTESIAN_POINT('',(5.39169646780806,-1.9,5.58578643762691));
#21571=CARTESIAN_POINT('Origin',(5.55669646780806,-1.9,8.4142135623731));
#21572=CARTESIAN_POINT('',(5.39169646780806,-1.8,8.4142135623731));
#21573=CARTESIAN_POINT('Origin',(5.55669646780806,-1.8,8.4142135623731));
#21574=CARTESIAN_POINT('',(5.39169646780806,-1.9,8.4142135623731));
#21575=CARTESIAN_POINT('Origin',(8.38512359255425,-1.9,8.4142135623731));
#21576=CARTESIAN_POINT('',(8.22012359255425,-1.8,8.4142135623731));
#21577=CARTESIAN_POINT('Origin',(8.38512359255425,-1.8,8.4142135623731));
#21578=CARTESIAN_POINT('',(8.22012359255425,-1.9,8.4142135623731));
#21579=CARTESIAN_POINT('Origin',(8.38512359255425,-1.9,5.58578643762691));
#21580=CARTESIAN_POINT('',(8.22012359255425,-1.8,5.58578643762691));
#21581=CARTESIAN_POINT('Origin',(8.38512359255425,-1.8,5.58578643762691));
#21582=CARTESIAN_POINT('',(8.22012359255425,-1.9,5.58578643762691));
#21583=CARTESIAN_POINT('Origin',(6.97091003018116,-1.9,7.));
#21584=CARTESIAN_POINT('',(5.37091003018116,-1.8,7.));
#21585=CARTESIAN_POINT('Origin',(6.97091003018116,-1.8,7.));
#21586=CARTESIAN_POINT('',(5.37091003018116,-1.9,7.));
#21587=CARTESIAN_POINT('Origin',(9.77091003018116,-1.,-0.1));
#21588=CARTESIAN_POINT('',(9.54591003018116,-1.,0.));
#21589=CARTESIAN_POINT('Origin',(9.77091003018116,-1.,0.));
#21590=CARTESIAN_POINT('',(9.54591003018116,-1.,0.8));
#21591=CARTESIAN_POINT('',(9.54591003018116,-1.,-0.1));
#21592=CARTESIAN_POINT('Origin',(9.77091003018116,-1.,0.8));
#21593=CARTESIAN_POINT('Origin',(4.17091003018116,1.,-0.1));
#21594=CARTESIAN_POINT('',(3.94591003018116,1.,0.));
#21595=CARTESIAN_POINT('Origin',(4.17091003018116,1.,0.));
#21596=CARTESIAN_POINT('',(3.94591003018116,1.,0.8));
#21597=CARTESIAN_POINT('',(3.94591003018116,1.,-0.1));
#21598=CARTESIAN_POINT('Origin',(4.17091003018116,1.,0.8));
#21599=CARTESIAN_POINT('Origin',(4.17091003018116,-1.,-0.1));
#21600=CARTESIAN_POINT('',(3.94591003018116,-1.,0.));
#21601=CARTESIAN_POINT('Origin',(4.17091003018116,-1.,0.));
#21602=CARTESIAN_POINT('',(3.94591003018116,-1.,0.8));
#21603=CARTESIAN_POINT('',(3.94591003018116,-1.,-0.1));
#21604=CARTESIAN_POINT('Origin',(4.17091003018116,-1.,0.8));
#21605=CARTESIAN_POINT('Origin',(9.77091003018116,1.,-0.1));
#21606=CARTESIAN_POINT('',(9.54591003018116,1.,0.));
#21607=CARTESIAN_POINT('Origin',(9.77091003018116,1.,0.));
#21608=CARTESIAN_POINT('',(9.54591003018116,1.,0.8));
#21609=CARTESIAN_POINT('',(9.54591003018116,1.,-0.1));
#21610=CARTESIAN_POINT('Origin',(9.77091003018116,1.,0.8));
#21611=CARTESIAN_POINT('Origin',(3.57091003018116,-1.8,0.8));
#21612=CARTESIAN_POINT('',(10.3709100301812,-1.8,0.8));
#21613=CARTESIAN_POINT('',(10.3709100301812,-1.8,0.8));
#21614=CARTESIAN_POINT('',(10.3709100301812,1.8,0.8));
#21615=CARTESIAN_POINT('',(10.3709100301812,-1.8,0.8));
#21616=CARTESIAN_POINT('',(10.3709100301812,1.8,0.8));
#21617=CARTESIAN_POINT('Origin',(3.57091003018116,-1.8,0.8));
#21618=CARTESIAN_POINT('',(4.77091003018116,1.8,0.8));
#21619=CARTESIAN_POINT('',(4.77091003018116,-1.8,0.8));
#21620=CARTESIAN_POINT('',(4.77091003018116,0.,0.8));
#21621=CARTESIAN_POINT('',(3.57091003018116,1.8,0.8));
#21622=CARTESIAN_POINT('',(10.3709100301812,1.8,0.8));
#21623=CARTESIAN_POINT('',(3.57091003018116,-1.8,0.8));
#21624=CARTESIAN_POINT('',(3.57091003018116,-1.8,0.8));
#21625=CARTESIAN_POINT('',(10.3709100301812,-1.8,0.8));
#21626=CARTESIAN_POINT('Origin',(3.57091003018116,-1.8,0.));
#21627=CARTESIAN_POINT('',(3.57091003018116,-1.8,0.));
#21628=CARTESIAN_POINT('',(3.57091003018116,-1.8,0.8));
#21629=CARTESIAN_POINT('',(3.57091003018116,1.8,0.));
#21630=CARTESIAN_POINT('',(3.57091003018116,1.8,0.8));
#21631=CARTESIAN_POINT('',(3.57091003018116,-1.8,0.));
#21632=CARTESIAN_POINT('Origin',(10.3709100301812,-1.8,0.8));
#21633=CARTESIAN_POINT('',(10.3709100301812,-1.8,0.));
#21634=CARTESIAN_POINT('',(10.3709100301812,-1.8,0.));
#21635=CARTESIAN_POINT('',(10.3709100301812,1.8,0.));
#21636=CARTESIAN_POINT('',(10.3709100301812,-1.8,0.));
#21637=CARTESIAN_POINT('',(10.3709100301812,1.8,0.));
#21638=CARTESIAN_POINT('Origin',(4.77091003018116,-1.8,0.));
#21639=CARTESIAN_POINT('',(4.77091003018116,-1.8,0.));
#21640=CARTESIAN_POINT('',(3.57091003018116,-1.8,0.));
#21641=CARTESIAN_POINT('Origin',(9.17091003018116,1.8,0.));
#21642=CARTESIAN_POINT('',(3.57091003018116,1.8,0.));
#21643=CARTESIAN_POINT('',(4.77091003018116,1.8,0.));
#21644=CARTESIAN_POINT('Origin',(4.77091003018116,1.8,0.));
#21645=CARTESIAN_POINT('Origin',(6.97091003018116,0.,0.));
#26925=UNCERTAINTY_MEASURE_WITH_UNIT(LENGTH_MEASURE(0.001),#27070,
'DISTANCE_ACCURACY_VALUE',
'Maximum model space distance between geometric entities at asserted c
onnectivities');
#26992=UNCERTAINTY_MEASURE_WITH_UNIT(LENGTH_MEASURE(0.001),#27070,
'DISTANCE_ACCURACY_VALUE',
'Maximum model space distance between geometric entities at asserted c
onnectivities');
#27002=(
GEOMETRIC_REPRESENTATION_CONTEXT(3)
GLOBAL_UNCERTAINTY_ASSIGNED_CONTEXT((#26925))
GLOBAL_UNIT_ASSIGNED_CONTEXT((#27070,#27072,#27073))
REPRESENTATION_CONTEXT('','3D')
);
#27069=(
GEOMETRIC_REPRESENTATION_CONTEXT(3)
GLOBAL_UNCERTAINTY_ASSIGNED_CONTEXT((#26992))
GLOBAL_UNIT_ASSIGNED_CONTEXT((#27070,#27072,#27073))
REPRESENTATION_CONTEXT('','3D')
);
#27070=(
LENGTH_UNIT()
NAMED_UNIT(*)
SI_UNIT(.CENTI.,.METRE.)
);
#27072=(
NAMED_UNIT(*)
PLANE_ANGLE_UNIT()
SI_UNIT($,.RADIAN.)
);
#27073=(
NAMED_UNIT(*)
SI_UNIT($,.STERADIAN.)
SOLID_ANGLE_UNIT()
);
#27083=SHAPE_DEFINITION_REPRESENTATION(#27159,#27360);
#27159=PRODUCT_DEFINITION_SHAPE('',$,#27437);
#27360=SHAPE_REPRESENTATION('',(#14792),#27002);
#27427=PRODUCT_DEFINITION_CONTEXT('part definition',#27657,'design');
#27437=PRODUCT_DEFINITION('Sliding bearing block',
'Sliding bearing block',#27513,#27427);
#27513=PRODUCT_DEFINITION_FORMATION('',$,#27668);
#27657=APPLICATION_CONTEXT(
'Core Data for Automotive Mechanical Design Process');
#27658=PRODUCT_CONTEXT('part definition',#27657,'mechanical');
#27668=PRODUCT('Sliding bearing block','Sliding bearing block',
'Sliding bearing block',(#27658));
#27791=COLOUR_RGB('Grey',0.48,0.52,0.57);
#27792=FILL_AREA_STYLE_COLOUR('',#27791);
#27793=FILL_AREA_STYLE('',(#27792));
#27794=SURFACE_STYLE_FILL_AREA(#27793);
#27795=SURFACE_SIDE_STYLE('',(#27794));
#27796=SURFACE_STYLE_USAGE(.BOTH.,#27795);
#27797=PRESENTATION_STYLE_ASSIGNMENT((#27796));
ENDSEC;
END-ISO-10303-21;
